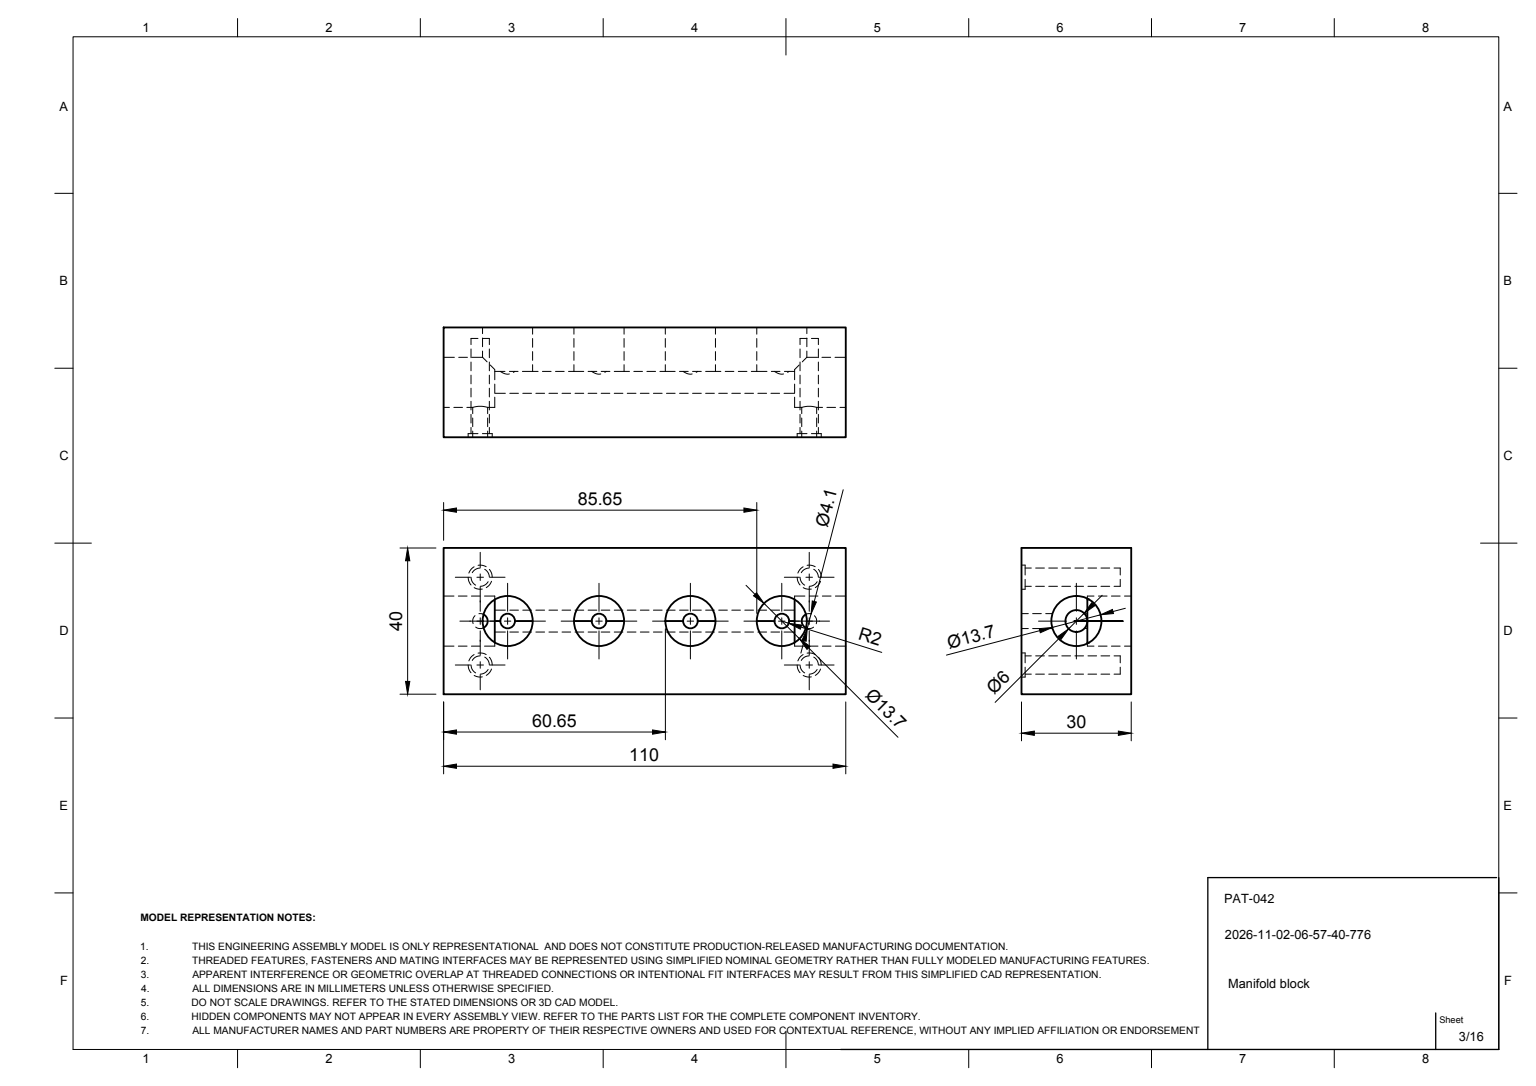
ISO-10303-21;
HEADER;
/* Generated by software containing ST-Developer
 * from STEP Tools, Inc. (www.steptools.com) 
 */

FILE_DESCRIPTION(
/* description */ ('Manifold and mounting hardware'),
/* implementation_level */ '2;1');

FILE_NAME(
/* name */ 'Manifold block.step',
/* time_stamp */ '2026-10-28T21:46:49-07:00',
/* author */ (''),
/* organization */ (''),
/* preprocessor_version */ 'ST-DEVELOPER v20.2',
/* originating_system */ 'Autodesk Translation Framework v15.17.0.0',
/* authorisation */ '');

FILE_SCHEMA (('AUTOMOTIVE_DESIGN { 1 0 10303 214 3 1 1 }'));
ENDSEC;

DATA;
#10=MECHANICAL_DESIGN_GEOMETRIC_PRESENTATION_REPRESENTATION('',(#150),#5638);
#122=SHAPE_REPRESENTATION_RELATIONSHIP('SRR','None',#5701,#136);
#136=ADVANCED_BREP_SHAPE_REPRESENTATION('',(#164),#5623);
#150=STYLED_ITEM('',(#5839),#164);
#164=MANIFOLD_SOLID_BREP('Body1',#3140);
#178=FACE_BOUND('',#528,.T.);
#179=FACE_BOUND('',#531,.T.);
#180=FACE_BOUND('',#539,.T.);
#181=FACE_BOUND('',#542,.T.);
#182=FACE_BOUND('',#545,.T.);
#183=FACE_BOUND('',#546,.T.);
#184=FACE_BOUND('',#555,.T.);
#185=FACE_BOUND('',#558,.T.);
#186=FACE_BOUND('',#560,.T.);
#187=FACE_BOUND('',#561,.T.);
#188=FACE_BOUND('',#562,.T.);
#189=FACE_BOUND('',#563,.T.);
#190=FACE_BOUND('',#565,.T.);
#191=FACE_BOUND('',#566,.T.);
#192=FACE_BOUND('',#567,.T.);
#193=FACE_BOUND('',#568,.T.);
#194=FACE_BOUND('',#569,.T.);
#195=FACE_BOUND('',#570,.T.);
#253=B_SPLINE_CURVE_WITH_KNOTS('',3,(#4697,#4698,#4699,#4700,#4701,#4702,
#4703,#4704,#4705,#4706),.UNSPECIFIED.,.F.,.F.,(4,2,2,2,4),(0.,0.0777490769060827,
0.155498153812165,0.233224303462309,0.310950453112452),.UNSPECIFIED.);
#254=B_SPLINE_CURVE_WITH_KNOTS('',3,(#4707,#4708,#4709,#4710,#4711,#4712,
#4713,#4714,#4715,#4716,#4717,#4718,#4719,#4720,#4721,#4722,#4723,#4724,
#4725,#4726,#4727,#4728,#4729,#4730,#4731,#4732),.UNSPECIFIED.,.F.,.F.,
(4,2,2,2,2,2,2,2,2,2,2,2,4),(0.310950453112452,0.388676602762596,0.466402752412739,
0.544151829318822,0.621900906224905,0.699649983130987,0.77739906003707,
0.855125209687213,0.932851359337357,1.0105775089875,1.08830365863764,1.16605273554373,
1.24380181244981),.UNSPECIFIED.);
#255=B_SPLINE_CURVE_WITH_KNOTS('',3,(#4767,#4768,#4769,#4770,#4771,#4772,
#4773,#4774,#4775,#4776),.UNSPECIFIED.,.F.,.F.,(4,2,2,2,4),(0.,0.0777490769060827,
0.155498153812165,0.233224303462309,0.310950453112452),.UNSPECIFIED.);
#256=B_SPLINE_CURVE_WITH_KNOTS('',3,(#4777,#4778,#4779,#4780,#4781,#4782,
#4783,#4784,#4785,#4786,#4787,#4788,#4789,#4790,#4791,#4792,#4793,#4794,
#4795,#4796,#4797,#4798,#4799,#4800,#4801,#4802),.UNSPECIFIED.,.F.,.F.,
(4,2,2,2,2,2,2,2,2,2,2,2,4),(0.310950453112452,0.388676602762596,0.466402752412739,
0.544151829318822,0.621900906224905,0.699649983130987,0.77739906003707,
0.855125209687213,0.932851359337357,1.0105775089875,1.08830365863764,1.16605273554373,
1.24380181244981),.UNSPECIFIED.);
#257=ELLIPSE('',#3314,0.96873629022557,0.685);
#258=ELLIPSE('',#3315,0.96873629022557,0.685);
#259=ELLIPSE('',#3316,0.96873629022557,0.685);
#260=ELLIPSE('',#3318,0.96873629022557,0.685);
#261=ELLIPSE('',#3325,0.96873629022557,0.685);
#262=ELLIPSE('',#3327,0.96873629022557,0.685);
#263=ELLIPSE('',#3329,0.96873629022557,0.685);
#264=ELLIPSE('',#3330,0.96873629022557,0.685);
#265=ELLIPSE('',#3371,0.96873629022557,0.685);
#266=ELLIPSE('',#3372,0.96873629022557,0.685);
#267=ELLIPSE('',#3373,0.96873629022557,0.685);
#268=ELLIPSE('',#3374,0.96873629022557,0.685);
#269=ELLIPSE('',#3376,0.96873629022557,0.685);
#270=ELLIPSE('',#3377,0.96873629022557,0.685);
#271=ELLIPSE('',#3378,0.96873629022557,0.685);
#272=ELLIPSE('',#3379,0.96873629022557,0.685);
#273=CYLINDRICAL_SURFACE('',#3313,0.685);
#274=CYLINDRICAL_SURFACE('',#3324,0.685);
#275=CYLINDRICAL_SURFACE('',#3332,0.205);
#276=CYLINDRICAL_SURFACE('',#3334,0.25);
#277=CYLINDRICAL_SURFACE('',#3338,0.25);
#278=CYLINDRICAL_SURFACE('',#3342,0.33);
#279=CYLINDRICAL_SURFACE('',#3346,0.33);
#280=CYLINDRICAL_SURFACE('',#3350,0.205);
#281=CYLINDRICAL_SURFACE('',#3352,0.25);
#282=CYLINDRICAL_SURFACE('',#3356,0.25);
#283=CYLINDRICAL_SURFACE('',#3360,0.33);
#284=CYLINDRICAL_SURFACE('',#3364,0.33);
#285=CYLINDRICAL_SURFACE('',#3369,0.685);
#286=CYLINDRICAL_SURFACE('',#3382,0.685);
#287=CYLINDRICAL_SURFACE('',#3386,0.685);
#330=FACE_OUTER_BOUND('',#516,.T.);
#331=FACE_OUTER_BOUND('',#517,.T.);
#332=FACE_OUTER_BOUND('',#518,.T.);
#333=FACE_OUTER_BOUND('',#519,.T.);
#334=FACE_OUTER_BOUND('',#520,.T.);
#335=FACE_OUTER_BOUND('',#521,.T.);
#336=FACE_OUTER_BOUND('',#522,.T.);
#337=FACE_OUTER_BOUND('',#523,.T.);
#338=FACE_OUTER_BOUND('',#524,.T.);
#339=FACE_OUTER_BOUND('',#525,.T.);
#340=FACE_OUTER_BOUND('',#526,.T.);
#341=FACE_OUTER_BOUND('',#527,.T.);
#342=FACE_OUTER_BOUND('',#529,.T.);
#343=FACE_OUTER_BOUND('',#530,.T.);
#344=FACE_OUTER_BOUND('',#532,.T.);
#345=FACE_OUTER_BOUND('',#533,.T.);
#346=FACE_OUTER_BOUND('',#534,.T.);
#347=FACE_OUTER_BOUND('',#535,.T.);
#348=FACE_OUTER_BOUND('',#536,.T.);
#349=FACE_OUTER_BOUND('',#537,.T.);
#350=FACE_OUTER_BOUND('',#538,.T.);
#351=FACE_OUTER_BOUND('',#540,.T.);
#352=FACE_OUTER_BOUND('',#541,.T.);
#353=FACE_OUTER_BOUND('',#543,.T.);
#354=FACE_OUTER_BOUND('',#544,.T.);
#355=FACE_OUTER_BOUND('',#547,.T.);
#356=FACE_OUTER_BOUND('',#548,.T.);
#357=FACE_OUTER_BOUND('',#549,.T.);
#358=FACE_OUTER_BOUND('',#550,.T.);
#359=FACE_OUTER_BOUND('',#551,.T.);
#360=FACE_OUTER_BOUND('',#552,.T.);
#361=FACE_OUTER_BOUND('',#553,.T.);
#362=FACE_OUTER_BOUND('',#554,.T.);
#363=FACE_OUTER_BOUND('',#556,.T.);
#364=FACE_OUTER_BOUND('',#557,.T.);
#365=FACE_OUTER_BOUND('',#559,.T.);
#366=FACE_OUTER_BOUND('',#564,.T.);
#516=EDGE_LOOP('',(#2044,#2045));
#517=EDGE_LOOP('',(#2046,#2047,#2048,#2049,#2050,#2051,#2052,#2053,#2054));
#518=EDGE_LOOP('',(#2055,#2056));
#519=EDGE_LOOP('',(#2057,#2058));
#520=EDGE_LOOP('',(#2059,#2060,#2061,#2062,#2063,#2064,#2065,#2066,#2067));
#521=EDGE_LOOP('',(#2068,#2069,#2070,#2071,#2072));
#522=EDGE_LOOP('',(#2073,#2074,#2075,#2076));
#523=EDGE_LOOP('',(#2077));
#524=EDGE_LOOP('',(#2078,#2079,#2080,#2081));
#525=EDGE_LOOP('',(#2082));
#526=EDGE_LOOP('',(#2083,#2084,#2085,#2086));
#527=EDGE_LOOP('',(#2087));
#528=EDGE_LOOP('',(#2088));
#529=EDGE_LOOP('',(#2089,#2090,#2091,#2092));
#530=EDGE_LOOP('',(#2093));
#531=EDGE_LOOP('',(#2094));
#532=EDGE_LOOP('',(#2095,#2096,#2097,#2098,#2099));
#533=EDGE_LOOP('',(#2100,#2101,#2102,#2103));
#534=EDGE_LOOP('',(#2104));
#535=EDGE_LOOP('',(#2105,#2106,#2107,#2108));
#536=EDGE_LOOP('',(#2109));
#537=EDGE_LOOP('',(#2110,#2111,#2112,#2113));
#538=EDGE_LOOP('',(#2114));
#539=EDGE_LOOP('',(#2115));
#540=EDGE_LOOP('',(#2116,#2117,#2118,#2119));
#541=EDGE_LOOP('',(#2120));
#542=EDGE_LOOP('',(#2121));
#543=EDGE_LOOP('',(#2122,#2123));
#544=EDGE_LOOP('',(#2124,#2125,#2126,#2127,#2128,#2129,#2130,#2131,#2132,
#2133,#2134,#2135,#2136,#2137,#2138,#2139,#2140,#2141,#2142,#2143,#2144,
#2145,#2146,#2147,#2148,#2149,#2150,#2151,#2152,#2153,#2154,#2155,#2156,
#2157,#2158,#2159));
#545=EDGE_LOOP('',(#2160,#2161));
#546=EDGE_LOOP('',(#2162,#2163));
#547=EDGE_LOOP('',(#2164,#2165));
#548=EDGE_LOOP('',(#2166,#2167,#2168,#2169,#2170,#2171,#2172,#2173,#2174));
#549=EDGE_LOOP('',(#2175,#2176));
#550=EDGE_LOOP('',(#2177,#2178,#2179,#2180,#2181,#2182,#2183,#2184,#2185));
#551=EDGE_LOOP('',(#2186,#2187));
#552=EDGE_LOOP('',(#2188,#2189));
#553=EDGE_LOOP('',(#2190,#2191,#2192,#2193));
#554=EDGE_LOOP('',(#2194,#2195,#2196,#2197));
#555=EDGE_LOOP('',(#2198));
#556=EDGE_LOOP('',(#2199,#2200,#2201,#2202));
#557=EDGE_LOOP('',(#2203,#2204,#2205,#2206));
#558=EDGE_LOOP('',(#2207));
#559=EDGE_LOOP('',(#2208,#2209,#2210,#2211));
#560=EDGE_LOOP('',(#2212));
#561=EDGE_LOOP('',(#2213));
#562=EDGE_LOOP('',(#2214));
#563=EDGE_LOOP('',(#2215));
#564=EDGE_LOOP('',(#2216,#2217,#2218,#2219));
#565=EDGE_LOOP('',(#2220));
#566=EDGE_LOOP('',(#2221));
#567=EDGE_LOOP('',(#2222));
#568=EDGE_LOOP('',(#2223));
#569=EDGE_LOOP('',(#2224));
#570=EDGE_LOOP('',(#2225));
#777=CIRCLE('',#3312,0.685);
#778=CIRCLE('',#3317,0.685);
#779=CIRCLE('',#3319,0.685);
#780=CIRCLE('',#3321,0.685);
#781=CIRCLE('',#3323,0.685);
#782=CIRCLE('',#3326,0.685);
#783=CIRCLE('',#3328,0.685);
#784=CIRCLE('',#3331,0.685);
#785=CIRCLE('',#3333,0.205);
#786=CIRCLE('',#3335,0.25);
#787=CIRCLE('',#3336,0.25);
#788=CIRCLE('',#3339,0.25);
#789=CIRCLE('',#3340,0.25);
#790=CIRCLE('',#3343,0.33);
#791=CIRCLE('',#3344,0.33);
#792=CIRCLE('',#3347,0.33);
#793=CIRCLE('',#3348,0.33);
#794=CIRCLE('',#3351,0.205);
#795=CIRCLE('',#3353,0.25);
#796=CIRCLE('',#3354,0.25);
#797=CIRCLE('',#3357,0.25);
#798=CIRCLE('',#3358,0.25);
#799=CIRCLE('',#3361,0.33);
#800=CIRCLE('',#3362,0.33);
#801=CIRCLE('',#3365,0.33);
#802=CIRCLE('',#3366,0.33);
#803=CIRCLE('',#3370,0.685);
#804=CIRCLE('',#3375,0.685);
#805=CIRCLE('',#3381,0.685);
#806=CIRCLE('',#3383,0.685);
#807=CIRCLE('',#3385,0.685);
#808=CIRCLE('',#3387,0.685);
#897=LINE('',#4650,#1144);
#898=LINE('',#4660,#1145);
#899=LINE('',#4668,#1146);
#900=LINE('',#4673,#1147);
#901=LINE('',#4680,#1148);
#902=LINE('',#4695,#1149);
#903=LINE('',#4737,#1150);
#904=LINE('',#4744,#1151);
#905=LINE('',#4751,#1152);
#906=LINE('',#4758,#1153);
#907=LINE('',#4765,#1154);
#908=LINE('',#4807,#1155);
#909=LINE('',#4814,#1156);
#910=LINE('',#4821,#1157);
#911=LINE('',#4828,#1158);
#912=LINE('',#4832,#1159);
#913=LINE('',#4836,#1160);
#914=LINE('',#4837,#1161);
#915=LINE('',#4839,#1162);
#916=LINE('',#4843,#1163);
#917=LINE('',#4847,#1164);
#918=LINE('',#4851,#1165);
#919=LINE('',#4854,#1166);
#920=LINE('',#4856,#1167);
#921=LINE('',#4862,#1168);
#922=LINE('',#4867,#1169);
#923=LINE('',#4873,#1170);
#924=LINE('',#4880,#1171);
#925=LINE('',#4882,#1172);
#926=LINE('',#4884,#1173);
#927=LINE('',#4885,#1174);
#928=LINE('',#4888,#1175);
#929=LINE('',#4890,#1176);
#930=LINE('',#4891,#1177);
#931=LINE('',#4894,#1178);
#932=LINE('',#4896,#1179);
#933=LINE('',#4897,#1180);
#934=LINE('',#4899,#1181);
#935=LINE('',#4900,#1182);
#1144=VECTOR('',#3678,1.);
#1145=VECTOR('',#3689,0.685);
#1146=VECTOR('',#3698,1.);
#1147=VECTOR('',#3703,1.);
#1148=VECTOR('',#3710,0.685);
#1149=VECTOR('',#3727,0.205);
#1150=VECTOR('',#3732,0.25);
#1151=VECTOR('',#3741,0.25);
#1152=VECTOR('',#3750,0.33);
#1153=VECTOR('',#3759,0.33);
#1154=VECTOR('',#3768,0.205);
#1155=VECTOR('',#3773,0.25);
#1156=VECTOR('',#3782,0.25);
#1157=VECTOR('',#3791,0.33);
#1158=VECTOR('',#3800,0.33);
#1159=VECTOR('',#3807,1.);
#1160=VECTOR('',#3812,0.685);
#1161=VECTOR('',#3813,1.);
#1162=VECTOR('',#3814,0.685);
#1163=VECTOR('',#3817,1.);
#1164=VECTOR('',#3820,0.685);
#1165=VECTOR('',#3823,1.);
#1166=VECTOR('',#3826,0.685);
#1167=VECTOR('',#3827,0.685);
#1168=VECTOR('',#3838,1.);
#1169=VECTOR('',#3845,0.685);
#1170=VECTOR('',#3854,0.685);
#1171=VECTOR('',#3863,1.);
#1172=VECTOR('',#3864,1.);
#1173=VECTOR('',#3865,1.);
#1174=VECTOR('',#3866,1.);
#1175=VECTOR('',#3869,1.);
#1176=VECTOR('',#3870,1.);
#1177=VECTOR('',#3871,1.);
#1178=VECTOR('',#3874,1.);
#1179=VECTOR('',#3875,1.);
#1180=VECTOR('',#3876,1.);
#1181=VECTOR('',#3879,1.);
#1182=VECTOR('',#3880,1.);
#1391=VERTEX_POINT('',#4648);
#1392=VERTEX_POINT('',#4649);
#1393=VERTEX_POINT('',#4653);
#1394=VERTEX_POINT('',#4654);
#1395=VERTEX_POINT('',#4657);
#1396=VERTEX_POINT('',#4659);
#1397=VERTEX_POINT('',#4662);
#1398=VERTEX_POINT('',#4666);
#1399=VERTEX_POINT('',#4667);
#1400=VERTEX_POINT('',#4671);
#1401=VERTEX_POINT('',#4672);
#1402=VERTEX_POINT('',#4676);
#1403=VERTEX_POINT('',#4677);
#1404=VERTEX_POINT('',#4679);
#1405=VERTEX_POINT('',#4682);
#1406=VERTEX_POINT('',#4684);
#1407=VERTEX_POINT('',#4686);
#1408=VERTEX_POINT('',#4688);
#1409=VERTEX_POINT('',#4692);
#1410=VERTEX_POINT('',#4694);
#1411=VERTEX_POINT('',#4696);
#1412=VERTEX_POINT('',#4734);
#1413=VERTEX_POINT('',#4736);
#1414=VERTEX_POINT('',#4741);
#1415=VERTEX_POINT('',#4743);
#1416=VERTEX_POINT('',#4748);
#1417=VERTEX_POINT('',#4750);
#1418=VERTEX_POINT('',#4755);
#1419=VERTEX_POINT('',#4757);
#1420=VERTEX_POINT('',#4762);
#1421=VERTEX_POINT('',#4764);
#1422=VERTEX_POINT('',#4766);
#1423=VERTEX_POINT('',#4804);
#1424=VERTEX_POINT('',#4806);
#1425=VERTEX_POINT('',#4811);
#1426=VERTEX_POINT('',#4813);
#1427=VERTEX_POINT('',#4818);
#1428=VERTEX_POINT('',#4820);
#1429=VERTEX_POINT('',#4825);
#1430=VERTEX_POINT('',#4827);
#1431=VERTEX_POINT('',#4834);
#1432=VERTEX_POINT('',#4838);
#1433=VERTEX_POINT('',#4840);
#1434=VERTEX_POINT('',#4842);
#1435=VERTEX_POINT('',#4844);
#1436=VERTEX_POINT('',#4846);
#1437=VERTEX_POINT('',#4848);
#1438=VERTEX_POINT('',#4850);
#1439=VERTEX_POINT('',#4852);
#1440=VERTEX_POINT('',#4855);
#1441=VERTEX_POINT('',#4866);
#1442=VERTEX_POINT('',#4872);
#1443=VERTEX_POINT('',#4878);
#1444=VERTEX_POINT('',#4879);
#1445=VERTEX_POINT('',#4881);
#1446=VERTEX_POINT('',#4883);
#1447=VERTEX_POINT('',#4887);
#1448=VERTEX_POINT('',#4889);
#1449=VERTEX_POINT('',#4893);
#1450=VERTEX_POINT('',#4895);
#1651=EDGE_CURVE('',#1391,#1392,#897,.T.);
#1652=EDGE_CURVE('',#1392,#1391,#777,.T.);
#1653=EDGE_CURVE('',#1393,#1394,#257,.T.);
#1654=EDGE_CURVE('',#1394,#1391,#258,.T.);
#1655=EDGE_CURVE('',#1392,#1395,#259,.T.);
#1656=EDGE_CURVE('',#1395,#1396,#898,.T.);
#1657=EDGE_CURVE('',#1396,#1396,#778,.T.);
#1658=EDGE_CURVE('',#1395,#1397,#260,.T.);
#1659=EDGE_CURVE('',#1393,#1397,#779,.T.);
#1660=EDGE_CURVE('',#1398,#1399,#899,.T.);
#1661=EDGE_CURVE('',#1399,#1398,#780,.T.);
#1662=EDGE_CURVE('',#1400,#1401,#900,.T.);
#1663=EDGE_CURVE('',#1401,#1400,#781,.T.);
#1664=EDGE_CURVE('',#1402,#1403,#261,.T.);
#1665=EDGE_CURVE('',#1403,#1404,#901,.T.);
#1666=EDGE_CURVE('',#1404,#1404,#782,.T.);
#1667=EDGE_CURVE('',#1403,#1405,#262,.T.);
#1668=EDGE_CURVE('',#1406,#1405,#783,.T.);
#1669=EDGE_CURVE('',#1406,#1407,#263,.T.);
#1670=EDGE_CURVE('',#1407,#1408,#264,.T.);
#1671=EDGE_CURVE('',#1402,#1408,#784,.T.);
#1672=EDGE_CURVE('',#1409,#1409,#785,.T.);
#1673=EDGE_CURVE('',#1409,#1410,#902,.T.);
#1674=EDGE_CURVE('',#1411,#1410,#253,.T.);
#1675=EDGE_CURVE('',#1410,#1411,#254,.T.);
#1676=EDGE_CURVE('',#1412,#1412,#786,.T.);
#1677=EDGE_CURVE('',#1412,#1413,#903,.T.);
#1678=EDGE_CURVE('',#1413,#1413,#787,.T.);
#1679=EDGE_CURVE('',#1414,#1414,#788,.T.);
#1680=EDGE_CURVE('',#1414,#1415,#904,.T.);
#1681=EDGE_CURVE('',#1415,#1415,#789,.T.);
#1682=EDGE_CURVE('',#1416,#1416,#790,.T.);
#1683=EDGE_CURVE('',#1416,#1417,#905,.T.);
#1684=EDGE_CURVE('',#1417,#1417,#791,.T.);
#1685=EDGE_CURVE('',#1418,#1418,#792,.T.);
#1686=EDGE_CURVE('',#1418,#1419,#906,.T.);
#1687=EDGE_CURVE('',#1419,#1419,#793,.T.);
#1688=EDGE_CURVE('',#1420,#1420,#794,.T.);
#1689=EDGE_CURVE('',#1420,#1421,#907,.T.);
#1690=EDGE_CURVE('',#1422,#1421,#255,.T.);
#1691=EDGE_CURVE('',#1421,#1422,#256,.T.);
#1692=EDGE_CURVE('',#1423,#1423,#795,.T.);
#1693=EDGE_CURVE('',#1423,#1424,#908,.T.);
#1694=EDGE_CURVE('',#1424,#1424,#796,.T.);
#1695=EDGE_CURVE('',#1425,#1425,#797,.T.);
#1696=EDGE_CURVE('',#1425,#1426,#909,.T.);
#1697=EDGE_CURVE('',#1426,#1426,#798,.T.);
#1698=EDGE_CURVE('',#1427,#1427,#799,.T.);
#1699=EDGE_CURVE('',#1427,#1428,#910,.T.);
#1700=EDGE_CURVE('',#1428,#1428,#800,.T.);
#1701=EDGE_CURVE('',#1429,#1429,#801,.T.);
#1702=EDGE_CURVE('',#1429,#1430,#911,.T.);
#1703=EDGE_CURVE('',#1430,#1430,#802,.T.);
#1704=EDGE_CURVE('',#1397,#1393,#912,.T.);
#1705=EDGE_CURVE('',#1431,#1431,#803,.T.);
#1706=EDGE_CURVE('',#1431,#1403,#913,.T.);
#1707=EDGE_CURVE('',#1408,#1402,#914,.T.);
#1708=EDGE_CURVE('',#1407,#1432,#915,.T.);
#1709=EDGE_CURVE('',#1433,#1432,#265,.T.);
#1710=EDGE_CURVE('',#1434,#1433,#916,.T.);
#1711=EDGE_CURVE('',#1435,#1434,#266,.T.);
#1712=EDGE_CURVE('',#1435,#1436,#917,.T.);
#1713=EDGE_CURVE('',#1437,#1436,#267,.T.);
#1714=EDGE_CURVE('',#1438,#1437,#918,.T.);
#1715=EDGE_CURVE('',#1439,#1438,#268,.T.);
#1716=EDGE_CURVE('',#1439,#1395,#919,.T.);
#1717=EDGE_CURVE('',#1394,#1440,#920,.T.);
#1718=EDGE_CURVE('',#1440,#1440,#804,.T.);
#1719=EDGE_CURVE('',#1399,#1439,#269,.T.);
#1720=EDGE_CURVE('',#1436,#1398,#270,.T.);
#1721=EDGE_CURVE('',#1401,#1435,#271,.T.);
#1722=EDGE_CURVE('',#1432,#1400,#272,.T.);
#1723=EDGE_CURVE('',#1405,#1406,#921,.T.);
#1724=EDGE_CURVE('',#1437,#1438,#805,.T.);
#1725=EDGE_CURVE('',#1436,#1441,#922,.T.);
#1726=EDGE_CURVE('',#1441,#1441,#806,.T.);
#1727=EDGE_CURVE('',#1433,#1434,#807,.T.);
#1728=EDGE_CURVE('',#1432,#1442,#923,.T.);
#1729=EDGE_CURVE('',#1442,#1442,#808,.T.);
#1730=EDGE_CURVE('',#1443,#1444,#924,.T.);
#1731=EDGE_CURVE('',#1444,#1445,#925,.T.);
#1732=EDGE_CURVE('',#1446,#1445,#926,.T.);
#1733=EDGE_CURVE('',#1443,#1446,#927,.T.);
#1734=EDGE_CURVE('',#1447,#1443,#928,.T.);
#1735=EDGE_CURVE('',#1448,#1446,#929,.T.);
#1736=EDGE_CURVE('',#1447,#1448,#930,.T.);
#1737=EDGE_CURVE('',#1449,#1447,#931,.T.);
#1738=EDGE_CURVE('',#1450,#1448,#932,.T.);
#1739=EDGE_CURVE('',#1449,#1450,#933,.T.);
#1740=EDGE_CURVE('',#1444,#1449,#934,.T.);
#1741=EDGE_CURVE('',#1445,#1450,#935,.T.);
#2044=ORIENTED_EDGE('',*,*,#1651,.T.);
#2045=ORIENTED_EDGE('',*,*,#1652,.T.);
#2046=ORIENTED_EDGE('',*,*,#1653,.T.);
#2047=ORIENTED_EDGE('',*,*,#1654,.T.);
#2048=ORIENTED_EDGE('',*,*,#1652,.F.);
#2049=ORIENTED_EDGE('',*,*,#1655,.T.);
#2050=ORIENTED_EDGE('',*,*,#1656,.T.);
#2051=ORIENTED_EDGE('',*,*,#1657,.F.);
#2052=ORIENTED_EDGE('',*,*,#1656,.F.);
#2053=ORIENTED_EDGE('',*,*,#1658,.T.);
#2054=ORIENTED_EDGE('',*,*,#1659,.F.);
#2055=ORIENTED_EDGE('',*,*,#1660,.T.);
#2056=ORIENTED_EDGE('',*,*,#1661,.T.);
#2057=ORIENTED_EDGE('',*,*,#1662,.T.);
#2058=ORIENTED_EDGE('',*,*,#1663,.T.);
#2059=ORIENTED_EDGE('',*,*,#1664,.T.);
#2060=ORIENTED_EDGE('',*,*,#1665,.T.);
#2061=ORIENTED_EDGE('',*,*,#1666,.F.);
#2062=ORIENTED_EDGE('',*,*,#1665,.F.);
#2063=ORIENTED_EDGE('',*,*,#1667,.T.);
#2064=ORIENTED_EDGE('',*,*,#1668,.F.);
#2065=ORIENTED_EDGE('',*,*,#1669,.T.);
#2066=ORIENTED_EDGE('',*,*,#1670,.T.);
#2067=ORIENTED_EDGE('',*,*,#1671,.F.);
#2068=ORIENTED_EDGE('',*,*,#1672,.F.);
#2069=ORIENTED_EDGE('',*,*,#1673,.T.);
#2070=ORIENTED_EDGE('',*,*,#1674,.F.);
#2071=ORIENTED_EDGE('',*,*,#1675,.F.);
#2072=ORIENTED_EDGE('',*,*,#1673,.F.);
#2073=ORIENTED_EDGE('',*,*,#1676,.F.);
#2074=ORIENTED_EDGE('',*,*,#1677,.T.);
#2075=ORIENTED_EDGE('',*,*,#1678,.T.);
#2076=ORIENTED_EDGE('',*,*,#1677,.F.);
#2077=ORIENTED_EDGE('',*,*,#1678,.F.);
#2078=ORIENTED_EDGE('',*,*,#1679,.F.);
#2079=ORIENTED_EDGE('',*,*,#1680,.T.);
#2080=ORIENTED_EDGE('',*,*,#1681,.T.);
#2081=ORIENTED_EDGE('',*,*,#1680,.F.);
#2082=ORIENTED_EDGE('',*,*,#1681,.F.);
#2083=ORIENTED_EDGE('',*,*,#1682,.F.);
#2084=ORIENTED_EDGE('',*,*,#1683,.T.);
#2085=ORIENTED_EDGE('',*,*,#1684,.T.);
#2086=ORIENTED_EDGE('',*,*,#1683,.F.);
#2087=ORIENTED_EDGE('',*,*,#1684,.F.);
#2088=ORIENTED_EDGE('',*,*,#1676,.T.);
#2089=ORIENTED_EDGE('',*,*,#1685,.F.);
#2090=ORIENTED_EDGE('',*,*,#1686,.T.);
#2091=ORIENTED_EDGE('',*,*,#1687,.T.);
#2092=ORIENTED_EDGE('',*,*,#1686,.F.);
#2093=ORIENTED_EDGE('',*,*,#1687,.F.);
#2094=ORIENTED_EDGE('',*,*,#1679,.T.);
#2095=ORIENTED_EDGE('',*,*,#1688,.F.);
#2096=ORIENTED_EDGE('',*,*,#1689,.T.);
#2097=ORIENTED_EDGE('',*,*,#1690,.F.);
#2098=ORIENTED_EDGE('',*,*,#1691,.F.);
#2099=ORIENTED_EDGE('',*,*,#1689,.F.);
#2100=ORIENTED_EDGE('',*,*,#1692,.F.);
#2101=ORIENTED_EDGE('',*,*,#1693,.T.);
#2102=ORIENTED_EDGE('',*,*,#1694,.T.);
#2103=ORIENTED_EDGE('',*,*,#1693,.F.);
#2104=ORIENTED_EDGE('',*,*,#1694,.F.);
#2105=ORIENTED_EDGE('',*,*,#1695,.F.);
#2106=ORIENTED_EDGE('',*,*,#1696,.T.);
#2107=ORIENTED_EDGE('',*,*,#1697,.T.);
#2108=ORIENTED_EDGE('',*,*,#1696,.F.);
#2109=ORIENTED_EDGE('',*,*,#1697,.F.);
#2110=ORIENTED_EDGE('',*,*,#1698,.F.);
#2111=ORIENTED_EDGE('',*,*,#1699,.T.);
#2112=ORIENTED_EDGE('',*,*,#1700,.T.);
#2113=ORIENTED_EDGE('',*,*,#1699,.F.);
#2114=ORIENTED_EDGE('',*,*,#1700,.F.);
#2115=ORIENTED_EDGE('',*,*,#1692,.T.);
#2116=ORIENTED_EDGE('',*,*,#1701,.F.);
#2117=ORIENTED_EDGE('',*,*,#1702,.T.);
#2118=ORIENTED_EDGE('',*,*,#1703,.T.);
#2119=ORIENTED_EDGE('',*,*,#1702,.F.);
#2120=ORIENTED_EDGE('',*,*,#1703,.F.);
#2121=ORIENTED_EDGE('',*,*,#1695,.T.);
#2122=ORIENTED_EDGE('',*,*,#1704,.T.);
#2123=ORIENTED_EDGE('',*,*,#1659,.T.);
#2124=ORIENTED_EDGE('',*,*,#1705,.F.);
#2125=ORIENTED_EDGE('',*,*,#1706,.T.);
#2126=ORIENTED_EDGE('',*,*,#1664,.F.);
#2127=ORIENTED_EDGE('',*,*,#1707,.F.);
#2128=ORIENTED_EDGE('',*,*,#1670,.F.);
#2129=ORIENTED_EDGE('',*,*,#1708,.T.);
#2130=ORIENTED_EDGE('',*,*,#1709,.F.);
#2131=ORIENTED_EDGE('',*,*,#1710,.F.);
#2132=ORIENTED_EDGE('',*,*,#1711,.F.);
#2133=ORIENTED_EDGE('',*,*,#1712,.T.);
#2134=ORIENTED_EDGE('',*,*,#1713,.F.);
#2135=ORIENTED_EDGE('',*,*,#1714,.F.);
#2136=ORIENTED_EDGE('',*,*,#1715,.F.);
#2137=ORIENTED_EDGE('',*,*,#1716,.T.);
#2138=ORIENTED_EDGE('',*,*,#1655,.F.);
#2139=ORIENTED_EDGE('',*,*,#1651,.F.);
#2140=ORIENTED_EDGE('',*,*,#1654,.F.);
#2141=ORIENTED_EDGE('',*,*,#1717,.T.);
#2142=ORIENTED_EDGE('',*,*,#1718,.F.);
#2143=ORIENTED_EDGE('',*,*,#1717,.F.);
#2144=ORIENTED_EDGE('',*,*,#1653,.F.);
#2145=ORIENTED_EDGE('',*,*,#1704,.F.);
#2146=ORIENTED_EDGE('',*,*,#1658,.F.);
#2147=ORIENTED_EDGE('',*,*,#1716,.F.);
#2148=ORIENTED_EDGE('',*,*,#1719,.F.);
#2149=ORIENTED_EDGE('',*,*,#1660,.F.);
#2150=ORIENTED_EDGE('',*,*,#1720,.F.);
#2151=ORIENTED_EDGE('',*,*,#1712,.F.);
#2152=ORIENTED_EDGE('',*,*,#1721,.F.);
#2153=ORIENTED_EDGE('',*,*,#1662,.F.);
#2154=ORIENTED_EDGE('',*,*,#1722,.F.);
#2155=ORIENTED_EDGE('',*,*,#1708,.F.);
#2156=ORIENTED_EDGE('',*,*,#1669,.F.);
#2157=ORIENTED_EDGE('',*,*,#1723,.F.);
#2158=ORIENTED_EDGE('',*,*,#1667,.F.);
#2159=ORIENTED_EDGE('',*,*,#1706,.F.);
#2160=ORIENTED_EDGE('',*,*,#1690,.T.);
#2161=ORIENTED_EDGE('',*,*,#1691,.T.);
#2162=ORIENTED_EDGE('',*,*,#1674,.T.);
#2163=ORIENTED_EDGE('',*,*,#1675,.T.);
#2164=ORIENTED_EDGE('',*,*,#1714,.T.);
#2165=ORIENTED_EDGE('',*,*,#1724,.T.);
#2166=ORIENTED_EDGE('',*,*,#1713,.T.);
#2167=ORIENTED_EDGE('',*,*,#1725,.T.);
#2168=ORIENTED_EDGE('',*,*,#1726,.F.);
#2169=ORIENTED_EDGE('',*,*,#1725,.F.);
#2170=ORIENTED_EDGE('',*,*,#1720,.T.);
#2171=ORIENTED_EDGE('',*,*,#1661,.F.);
#2172=ORIENTED_EDGE('',*,*,#1719,.T.);
#2173=ORIENTED_EDGE('',*,*,#1715,.T.);
#2174=ORIENTED_EDGE('',*,*,#1724,.F.);
#2175=ORIENTED_EDGE('',*,*,#1710,.T.);
#2176=ORIENTED_EDGE('',*,*,#1727,.T.);
#2177=ORIENTED_EDGE('',*,*,#1709,.T.);
#2178=ORIENTED_EDGE('',*,*,#1728,.T.);
#2179=ORIENTED_EDGE('',*,*,#1729,.F.);
#2180=ORIENTED_EDGE('',*,*,#1728,.F.);
#2181=ORIENTED_EDGE('',*,*,#1722,.T.);
#2182=ORIENTED_EDGE('',*,*,#1663,.F.);
#2183=ORIENTED_EDGE('',*,*,#1721,.T.);
#2184=ORIENTED_EDGE('',*,*,#1711,.T.);
#2185=ORIENTED_EDGE('',*,*,#1727,.F.);
#2186=ORIENTED_EDGE('',*,*,#1707,.T.);
#2187=ORIENTED_EDGE('',*,*,#1671,.T.);
#2188=ORIENTED_EDGE('',*,*,#1723,.T.);
#2189=ORIENTED_EDGE('',*,*,#1668,.T.);
#2190=ORIENTED_EDGE('',*,*,#1730,.T.);
#2191=ORIENTED_EDGE('',*,*,#1731,.T.);
#2192=ORIENTED_EDGE('',*,*,#1732,.F.);
#2193=ORIENTED_EDGE('',*,*,#1733,.F.);
#2194=ORIENTED_EDGE('',*,*,#1734,.T.);
#2195=ORIENTED_EDGE('',*,*,#1733,.T.);
#2196=ORIENTED_EDGE('',*,*,#1735,.F.);
#2197=ORIENTED_EDGE('',*,*,#1736,.F.);
#2198=ORIENTED_EDGE('',*,*,#1718,.T.);
#2199=ORIENTED_EDGE('',*,*,#1737,.T.);
#2200=ORIENTED_EDGE('',*,*,#1736,.T.);
#2201=ORIENTED_EDGE('',*,*,#1738,.F.);
#2202=ORIENTED_EDGE('',*,*,#1739,.F.);
#2203=ORIENTED_EDGE('',*,*,#1740,.T.);
#2204=ORIENTED_EDGE('',*,*,#1739,.T.);
#2205=ORIENTED_EDGE('',*,*,#1741,.F.);
#2206=ORIENTED_EDGE('',*,*,#1731,.F.);
#2207=ORIENTED_EDGE('',*,*,#1705,.T.);
#2208=ORIENTED_EDGE('',*,*,#1741,.T.);
#2209=ORIENTED_EDGE('',*,*,#1738,.T.);
#2210=ORIENTED_EDGE('',*,*,#1735,.T.);
#2211=ORIENTED_EDGE('',*,*,#1732,.T.);
#2212=ORIENTED_EDGE('',*,*,#1657,.T.);
#2213=ORIENTED_EDGE('',*,*,#1726,.T.);
#2214=ORIENTED_EDGE('',*,*,#1729,.T.);
#2215=ORIENTED_EDGE('',*,*,#1666,.T.);
#2216=ORIENTED_EDGE('',*,*,#1740,.F.);
#2217=ORIENTED_EDGE('',*,*,#1730,.F.);
#2218=ORIENTED_EDGE('',*,*,#1734,.F.);
#2219=ORIENTED_EDGE('',*,*,#1737,.F.);
#2220=ORIENTED_EDGE('',*,*,#1672,.T.);
#2221=ORIENTED_EDGE('',*,*,#1682,.T.);
#2222=ORIENTED_EDGE('',*,*,#1685,.T.);
#2223=ORIENTED_EDGE('',*,*,#1688,.T.);
#2224=ORIENTED_EDGE('',*,*,#1698,.T.);
#2225=ORIENTED_EDGE('',*,*,#1701,.T.);
#2830=PLANE('',#3311);
#2831=PLANE('',#3320);
#2832=PLANE('',#3322);
#2833=PLANE('',#3337);
#2834=PLANE('',#3341);
#2835=PLANE('',#3345);
#2836=PLANE('',#3349);
#2837=PLANE('',#3355);
#2838=PLANE('',#3359);
#2839=PLANE('',#3363);
#2840=PLANE('',#3367);
#2841=PLANE('',#3368);
#2842=PLANE('',#3380);
#2843=PLANE('',#3384);
#2844=PLANE('',#3388);
#2845=PLANE('',#3389);
#2846=PLANE('',#3390);
#2847=PLANE('',#3391);
#2848=PLANE('',#3392);
#2849=PLANE('',#3393);
#2850=PLANE('',#3394);
#2851=PLANE('',#3395);
#2954=ADVANCED_FACE('',(#330),#2830,.T.);
#2955=ADVANCED_FACE('',(#331),#273,.F.);
#2956=ADVANCED_FACE('',(#332),#2831,.T.);
#2957=ADVANCED_FACE('',(#333),#2832,.T.);
#2958=ADVANCED_FACE('',(#334),#274,.F.);
#2959=ADVANCED_FACE('',(#335),#275,.F.);
#2960=ADVANCED_FACE('',(#336),#276,.F.);
#2961=ADVANCED_FACE('',(#337),#2833,.F.);
#2962=ADVANCED_FACE('',(#338),#277,.F.);
#2963=ADVANCED_FACE('',(#339),#2834,.F.);
#2964=ADVANCED_FACE('',(#340),#278,.F.);
#2965=ADVANCED_FACE('',(#341,#178),#2835,.F.);
#2966=ADVANCED_FACE('',(#342),#279,.F.);
#2967=ADVANCED_FACE('',(#343,#179),#2836,.F.);
#2968=ADVANCED_FACE('',(#344),#280,.F.);
#2969=ADVANCED_FACE('',(#345),#281,.F.);
#2970=ADVANCED_FACE('',(#346),#2837,.F.);
#2971=ADVANCED_FACE('',(#347),#282,.F.);
#2972=ADVANCED_FACE('',(#348),#2838,.F.);
#2973=ADVANCED_FACE('',(#349),#283,.F.);
#2974=ADVANCED_FACE('',(#350,#180),#2839,.F.);
#2975=ADVANCED_FACE('',(#351),#284,.F.);
#2976=ADVANCED_FACE('',(#352,#181),#2840,.F.);
#2977=ADVANCED_FACE('',(#353),#2841,.T.);
#2978=ADVANCED_FACE('',(#354,#182,#183),#285,.F.);
#2979=ADVANCED_FACE('',(#355),#2842,.T.);
#2980=ADVANCED_FACE('',(#356),#286,.F.);
#2981=ADVANCED_FACE('',(#357),#2843,.T.);
#2982=ADVANCED_FACE('',(#358),#287,.F.);
#2983=ADVANCED_FACE('',(#359),#2844,.T.);
#2984=ADVANCED_FACE('',(#360),#2845,.T.);
#2985=ADVANCED_FACE('',(#361),#2846,.T.);
#2986=ADVANCED_FACE('',(#362,#184),#2847,.T.);
#2987=ADVANCED_FACE('',(#363),#2848,.T.);
#2988=ADVANCED_FACE('',(#364,#185),#2849,.T.);
#2989=ADVANCED_FACE('',(#365,#186,#187,#188,#189),#2850,.T.);
#2990=ADVANCED_FACE('',(#366,#190,#191,#192,#193,#194,#195),#2851,.F.);
#3140=CLOSED_SHELL('',(#2954,#2955,#2956,#2957,#2958,#2959,#2960,#2961,
#2962,#2963,#2964,#2965,#2966,#2967,#2968,#2969,#2970,#2971,#2972,#2973,
#2974,#2975,#2976,#2977,#2978,#2979,#2980,#2981,#2982,#2983,#2984,#2985,
#2986,#2987,#2988,#2989,#2990));
#3310=AXIS2_PLACEMENT_3D('',#4646,#3674,#3675);
#3311=AXIS2_PLACEMENT_3D('',#4647,#3676,#3677);
#3312=AXIS2_PLACEMENT_3D('',#4651,#3679,#3680);
#3313=AXIS2_PLACEMENT_3D('',#4652,#3681,#3682);
#3314=AXIS2_PLACEMENT_3D('',#4655,#3683,#3684);
#3315=AXIS2_PLACEMENT_3D('',#4656,#3685,#3686);
#3316=AXIS2_PLACEMENT_3D('',#4658,#3687,#3688);
#3317=AXIS2_PLACEMENT_3D('',#4661,#3690,#3691);
#3318=AXIS2_PLACEMENT_3D('',#4663,#3692,#3693);
#3319=AXIS2_PLACEMENT_3D('',#4664,#3694,#3695);
#3320=AXIS2_PLACEMENT_3D('',#4665,#3696,#3697);
#3321=AXIS2_PLACEMENT_3D('',#4669,#3699,#3700);
#3322=AXIS2_PLACEMENT_3D('',#4670,#3701,#3702);
#3323=AXIS2_PLACEMENT_3D('',#4674,#3704,#3705);
#3324=AXIS2_PLACEMENT_3D('',#4675,#3706,#3707);
#3325=AXIS2_PLACEMENT_3D('',#4678,#3708,#3709);
#3326=AXIS2_PLACEMENT_3D('',#4681,#3711,#3712);
#3327=AXIS2_PLACEMENT_3D('',#4683,#3713,#3714);
#3328=AXIS2_PLACEMENT_3D('',#4685,#3715,#3716);
#3329=AXIS2_PLACEMENT_3D('',#4687,#3717,#3718);
#3330=AXIS2_PLACEMENT_3D('',#4689,#3719,#3720);
#3331=AXIS2_PLACEMENT_3D('',#4690,#3721,#3722);
#3332=AXIS2_PLACEMENT_3D('',#4691,#3723,#3724);
#3333=AXIS2_PLACEMENT_3D('',#4693,#3725,#3726);
#3334=AXIS2_PLACEMENT_3D('',#4733,#3728,#3729);
#3335=AXIS2_PLACEMENT_3D('',#4735,#3730,#3731);
#3336=AXIS2_PLACEMENT_3D('',#4738,#3733,#3734);
#3337=AXIS2_PLACEMENT_3D('',#4739,#3735,#3736);
#3338=AXIS2_PLACEMENT_3D('',#4740,#3737,#3738);
#3339=AXIS2_PLACEMENT_3D('',#4742,#3739,#3740);
#3340=AXIS2_PLACEMENT_3D('',#4745,#3742,#3743);
#3341=AXIS2_PLACEMENT_3D('',#4746,#3744,#3745);
#3342=AXIS2_PLACEMENT_3D('',#4747,#3746,#3747);
#3343=AXIS2_PLACEMENT_3D('',#4749,#3748,#3749);
#3344=AXIS2_PLACEMENT_3D('',#4752,#3751,#3752);
#3345=AXIS2_PLACEMENT_3D('',#4753,#3753,#3754);
#3346=AXIS2_PLACEMENT_3D('',#4754,#3755,#3756);
#3347=AXIS2_PLACEMENT_3D('',#4756,#3757,#3758);
#3348=AXIS2_PLACEMENT_3D('',#4759,#3760,#3761);
#3349=AXIS2_PLACEMENT_3D('',#4760,#3762,#3763);
#3350=AXIS2_PLACEMENT_3D('',#4761,#3764,#3765);
#3351=AXIS2_PLACEMENT_3D('',#4763,#3766,#3767);
#3352=AXIS2_PLACEMENT_3D('',#4803,#3769,#3770);
#3353=AXIS2_PLACEMENT_3D('',#4805,#3771,#3772);
#3354=AXIS2_PLACEMENT_3D('',#4808,#3774,#3775);
#3355=AXIS2_PLACEMENT_3D('',#4809,#3776,#3777);
#3356=AXIS2_PLACEMENT_3D('',#4810,#3778,#3779);
#3357=AXIS2_PLACEMENT_3D('',#4812,#3780,#3781);
#3358=AXIS2_PLACEMENT_3D('',#4815,#3783,#3784);
#3359=AXIS2_PLACEMENT_3D('',#4816,#3785,#3786);
#3360=AXIS2_PLACEMENT_3D('',#4817,#3787,#3788);
#3361=AXIS2_PLACEMENT_3D('',#4819,#3789,#3790);
#3362=AXIS2_PLACEMENT_3D('',#4822,#3792,#3793);
#3363=AXIS2_PLACEMENT_3D('',#4823,#3794,#3795);
#3364=AXIS2_PLACEMENT_3D('',#4824,#3796,#3797);
#3365=AXIS2_PLACEMENT_3D('',#4826,#3798,#3799);
#3366=AXIS2_PLACEMENT_3D('',#4829,#3801,#3802);
#3367=AXIS2_PLACEMENT_3D('',#4830,#3803,#3804);
#3368=AXIS2_PLACEMENT_3D('',#4831,#3805,#3806);
#3369=AXIS2_PLACEMENT_3D('',#4833,#3808,#3809);
#3370=AXIS2_PLACEMENT_3D('',#4835,#3810,#3811);
#3371=AXIS2_PLACEMENT_3D('',#4841,#3815,#3816);
#3372=AXIS2_PLACEMENT_3D('',#4845,#3818,#3819);
#3373=AXIS2_PLACEMENT_3D('',#4849,#3821,#3822);
#3374=AXIS2_PLACEMENT_3D('',#4853,#3824,#3825);
#3375=AXIS2_PLACEMENT_3D('',#4857,#3828,#3829);
#3376=AXIS2_PLACEMENT_3D('',#4858,#3830,#3831);
#3377=AXIS2_PLACEMENT_3D('',#4859,#3832,#3833);
#3378=AXIS2_PLACEMENT_3D('',#4860,#3834,#3835);
#3379=AXIS2_PLACEMENT_3D('',#4861,#3836,#3837);
#3380=AXIS2_PLACEMENT_3D('',#4863,#3839,#3840);
#3381=AXIS2_PLACEMENT_3D('',#4864,#3841,#3842);
#3382=AXIS2_PLACEMENT_3D('',#4865,#3843,#3844);
#3383=AXIS2_PLACEMENT_3D('',#4868,#3846,#3847);
#3384=AXIS2_PLACEMENT_3D('',#4869,#3848,#3849);
#3385=AXIS2_PLACEMENT_3D('',#4870,#3850,#3851);
#3386=AXIS2_PLACEMENT_3D('',#4871,#3852,#3853);
#3387=AXIS2_PLACEMENT_3D('',#4874,#3855,#3856);
#3388=AXIS2_PLACEMENT_3D('',#4875,#3857,#3858);
#3389=AXIS2_PLACEMENT_3D('',#4876,#3859,#3860);
#3390=AXIS2_PLACEMENT_3D('',#4877,#3861,#3862);
#3391=AXIS2_PLACEMENT_3D('',#4886,#3867,#3868);
#3392=AXIS2_PLACEMENT_3D('',#4892,#3872,#3873);
#3393=AXIS2_PLACEMENT_3D('',#4898,#3877,#3878);
#3394=AXIS2_PLACEMENT_3D('',#4901,#3881,#3882);
#3395=AXIS2_PLACEMENT_3D('',#4902,#3883,#3884);
#3674=DIRECTION('axis',(0.,0.,1.));
#3675=DIRECTION('refdir',(1.,0.,0.));
#3676=DIRECTION('center_axis',(0.,0.,1.));
#3677=DIRECTION('ref_axis',(1.,0.,0.));
#3678=DIRECTION('',(-1.,0.,0.));
#3679=DIRECTION('center_axis',(0.,0.,1.));
#3680=DIRECTION('ref_axis',(1.,0.,0.));
#3681=DIRECTION('center_axis',(0.,0.,1.));
#3682=DIRECTION('ref_axis',(1.,0.,0.));
#3683=DIRECTION('center_axis',(0.707106781186548,0.,-0.707106781186547));
#3684=DIRECTION('ref_axis',(-0.707106781186547,0.,-0.707106781186548));
#3685=DIRECTION('center_axis',(0.707106781186548,0.,-0.707106781186547));
#3686=DIRECTION('ref_axis',(-0.707106781186547,0.,-0.707106781186548));
#3687=DIRECTION('center_axis',(-0.707106781186548,0.,-0.707106781186547));
#3688=DIRECTION('ref_axis',(0.707106781186547,0.,-0.707106781186548));
#3689=DIRECTION('',(0.,0.,1.));
#3690=DIRECTION('center_axis',(0.,0.,-1.));
#3691=DIRECTION('ref_axis',(1.,0.,0.));
#3692=DIRECTION('center_axis',(-0.707106781186548,0.,-0.707106781186547));
#3693=DIRECTION('ref_axis',(0.707106781186547,0.,-0.707106781186548));
#3694=DIRECTION('center_axis',(0.,0.,1.));
#3695=DIRECTION('ref_axis',(1.,0.,0.));
#3696=DIRECTION('center_axis',(0.,0.,1.));
#3697=DIRECTION('ref_axis',(1.,0.,0.));
#3698=DIRECTION('',(1.,0.,0.));
#3699=DIRECTION('center_axis',(0.,0.,1.));
#3700=DIRECTION('ref_axis',(1.,0.,0.));
#3701=DIRECTION('center_axis',(0.,0.,1.));
#3702=DIRECTION('ref_axis',(1.,0.,0.));
#3703=DIRECTION('',(1.,0.,0.));
#3704=DIRECTION('center_axis',(0.,0.,1.));
#3705=DIRECTION('ref_axis',(1.,0.,0.));
#3706=DIRECTION('center_axis',(0.,0.,1.));
#3707=DIRECTION('ref_axis',(1.,0.,0.));
#3708=DIRECTION('center_axis',(-0.707106781186548,0.,-0.707106781186548));
#3709=DIRECTION('ref_axis',(0.707106781186548,0.,-0.707106781186548));
#3710=DIRECTION('',(0.,0.,1.));
#3711=DIRECTION('center_axis',(0.,0.,-1.));
#3712=DIRECTION('ref_axis',(1.,0.,0.));
#3713=DIRECTION('center_axis',(-0.707106781186548,0.,-0.707106781186548));
#3714=DIRECTION('ref_axis',(0.707106781186548,0.,-0.707106781186548));
#3715=DIRECTION('center_axis',(0.,0.,1.));
#3716=DIRECTION('ref_axis',(1.,0.,0.));
#3717=DIRECTION('center_axis',(0.707106781186548,0.,-0.707106781186547));
#3718=DIRECTION('ref_axis',(-0.707106781186547,0.,-0.707106781186548));
#3719=DIRECTION('center_axis',(0.707106781186548,0.,-0.707106781186547));
#3720=DIRECTION('ref_axis',(-0.707106781186547,0.,-0.707106781186548));
#3721=DIRECTION('center_axis',(0.,0.,1.));
#3722=DIRECTION('ref_axis',(1.,0.,0.));
#3723=DIRECTION('center_axis',(0.,0.,1.));
#3724=DIRECTION('ref_axis',(1.,0.,0.));
#3725=DIRECTION('center_axis',(0.,0.,1.));
#3726=DIRECTION('ref_axis',(1.,0.,0.));
#3727=DIRECTION('',(0.,0.,1.));
#3728=DIRECTION('center_axis',(0.,0.,1.));
#3729=DIRECTION('ref_axis',(1.,0.,0.));
#3730=DIRECTION('center_axis',(0.,0.,1.));
#3731=DIRECTION('ref_axis',(1.,0.,0.));
#3732=DIRECTION('',(0.,0.,1.));
#3733=DIRECTION('center_axis',(0.,0.,1.));
#3734=DIRECTION('ref_axis',(1.,0.,0.));
#3735=DIRECTION('center_axis',(0.,0.,1.));
#3736=DIRECTION('ref_axis',(1.,0.,0.));
#3737=DIRECTION('center_axis',(0.,0.,1.));
#3738=DIRECTION('ref_axis',(1.,0.,0.));
#3739=DIRECTION('center_axis',(0.,0.,1.));
#3740=DIRECTION('ref_axis',(1.,0.,0.));
#3741=DIRECTION('',(0.,0.,1.));
#3742=DIRECTION('center_axis',(0.,0.,1.));
#3743=DIRECTION('ref_axis',(1.,0.,0.));
#3744=DIRECTION('center_axis',(0.,0.,1.));
#3745=DIRECTION('ref_axis',(1.,0.,0.));
#3746=DIRECTION('center_axis',(0.,0.,1.));
#3747=DIRECTION('ref_axis',(1.,0.,0.));
#3748=DIRECTION('center_axis',(0.,0.,1.));
#3749=DIRECTION('ref_axis',(1.,0.,0.));
#3750=DIRECTION('',(0.,0.,1.));
#3751=DIRECTION('center_axis',(0.,0.,1.));
#3752=DIRECTION('ref_axis',(1.,0.,0.));
#3753=DIRECTION('center_axis',(0.,0.,1.));
#3754=DIRECTION('ref_axis',(1.,0.,0.));
#3755=DIRECTION('center_axis',(0.,0.,1.));
#3756=DIRECTION('ref_axis',(1.,0.,0.));
#3757=DIRECTION('center_axis',(0.,0.,1.));
#3758=DIRECTION('ref_axis',(1.,0.,0.));
#3759=DIRECTION('',(0.,0.,1.));
#3760=DIRECTION('center_axis',(0.,0.,1.));
#3761=DIRECTION('ref_axis',(1.,0.,0.));
#3762=DIRECTION('center_axis',(0.,0.,1.));
#3763=DIRECTION('ref_axis',(1.,0.,0.));
#3764=DIRECTION('center_axis',(0.,0.,1.));
#3765=DIRECTION('ref_axis',(1.,0.,0.));
#3766=DIRECTION('center_axis',(0.,0.,1.));
#3767=DIRECTION('ref_axis',(1.,0.,0.));
#3768=DIRECTION('',(0.,0.,1.));
#3769=DIRECTION('center_axis',(0.,0.,1.));
#3770=DIRECTION('ref_axis',(1.,0.,0.));
#3771=DIRECTION('center_axis',(0.,0.,1.));
#3772=DIRECTION('ref_axis',(1.,0.,0.));
#3773=DIRECTION('',(0.,0.,1.));
#3774=DIRECTION('center_axis',(0.,0.,1.));
#3775=DIRECTION('ref_axis',(1.,0.,0.));
#3776=DIRECTION('center_axis',(0.,0.,1.));
#3777=DIRECTION('ref_axis',(1.,0.,0.));
#3778=DIRECTION('center_axis',(0.,0.,1.));
#3779=DIRECTION('ref_axis',(1.,0.,0.));
#3780=DIRECTION('center_axis',(0.,0.,1.));
#3781=DIRECTION('ref_axis',(1.,0.,0.));
#3782=DIRECTION('',(0.,0.,1.));
#3783=DIRECTION('center_axis',(0.,0.,1.));
#3784=DIRECTION('ref_axis',(1.,0.,0.));
#3785=DIRECTION('center_axis',(0.,0.,1.));
#3786=DIRECTION('ref_axis',(1.,0.,0.));
#3787=DIRECTION('center_axis',(0.,0.,1.));
#3788=DIRECTION('ref_axis',(1.,0.,0.));
#3789=DIRECTION('center_axis',(0.,0.,1.));
#3790=DIRECTION('ref_axis',(1.,0.,0.));
#3791=DIRECTION('',(0.,0.,1.));
#3792=DIRECTION('center_axis',(0.,0.,1.));
#3793=DIRECTION('ref_axis',(1.,0.,0.));
#3794=DIRECTION('center_axis',(0.,0.,1.));
#3795=DIRECTION('ref_axis',(1.,0.,0.));
#3796=DIRECTION('center_axis',(0.,0.,1.));
#3797=DIRECTION('ref_axis',(1.,0.,0.));
#3798=DIRECTION('center_axis',(0.,0.,1.));
#3799=DIRECTION('ref_axis',(1.,0.,0.));
#3800=DIRECTION('',(0.,0.,1.));
#3801=DIRECTION('center_axis',(0.,0.,1.));
#3802=DIRECTION('ref_axis',(1.,0.,0.));
#3803=DIRECTION('center_axis',(0.,0.,1.));
#3804=DIRECTION('ref_axis',(1.,0.,0.));
#3805=DIRECTION('center_axis',(0.,0.,1.));
#3806=DIRECTION('ref_axis',(1.,0.,0.));
#3807=DIRECTION('',(1.,0.,0.));
#3808=DIRECTION('center_axis',(1.,0.,0.));
#3809=DIRECTION('ref_axis',(0.,0.,-1.));
#3810=DIRECTION('center_axis',(1.,0.,0.));
#3811=DIRECTION('ref_axis',(0.,0.,-1.));
#3812=DIRECTION('',(1.,0.,0.));
#3813=DIRECTION('',(-1.,0.,0.));
#3814=DIRECTION('',(1.,0.,0.));
#3815=DIRECTION('center_axis',(-0.707106781186548,0.,-0.707106781186547));
#3816=DIRECTION('ref_axis',(0.707106781186547,0.,-0.707106781186548));
#3817=DIRECTION('',(-1.,0.,0.));
#3818=DIRECTION('center_axis',(0.707106781186548,0.,-0.707106781186547));
#3819=DIRECTION('ref_axis',(-0.707106781186547,0.,-0.707106781186548));
#3820=DIRECTION('',(1.,0.,0.));
#3821=DIRECTION('center_axis',(-0.707106781186548,0.,-0.707106781186547));
#3822=DIRECTION('ref_axis',(0.707106781186547,0.,-0.707106781186548));
#3823=DIRECTION('',(-1.,0.,0.));
#3824=DIRECTION('center_axis',(0.707106781186548,0.,-0.707106781186547));
#3825=DIRECTION('ref_axis',(-0.707106781186547,0.,-0.707106781186548));
#3826=DIRECTION('',(1.,0.,0.));
#3827=DIRECTION('',(1.,0.,0.));
#3828=DIRECTION('center_axis',(-1.,0.,0.));
#3829=DIRECTION('ref_axis',(0.,0.,-1.));
#3830=DIRECTION('center_axis',(0.707106781186548,0.,-0.707106781186547));
#3831=DIRECTION('ref_axis',(-0.707106781186547,0.,-0.707106781186548));
#3832=DIRECTION('center_axis',(-0.707106781186548,0.,-0.707106781186547));
#3833=DIRECTION('ref_axis',(0.707106781186547,0.,-0.707106781186548));
#3834=DIRECTION('center_axis',(0.707106781186548,0.,-0.707106781186547));
#3835=DIRECTION('ref_axis',(-0.707106781186547,0.,-0.707106781186548));
#3836=DIRECTION('center_axis',(-0.707106781186548,0.,-0.707106781186547));
#3837=DIRECTION('ref_axis',(0.707106781186547,0.,-0.707106781186548));
#3838=DIRECTION('',(1.,0.,0.));
#3839=DIRECTION('center_axis',(0.,0.,1.));
#3840=DIRECTION('ref_axis',(1.,0.,0.));
#3841=DIRECTION('center_axis',(0.,0.,1.));
#3842=DIRECTION('ref_axis',(1.,0.,0.));
#3843=DIRECTION('center_axis',(0.,0.,1.));
#3844=DIRECTION('ref_axis',(1.,0.,0.));
#3845=DIRECTION('',(0.,0.,1.));
#3846=DIRECTION('center_axis',(0.,0.,-1.));
#3847=DIRECTION('ref_axis',(1.,0.,0.));
#3848=DIRECTION('center_axis',(0.,0.,1.));
#3849=DIRECTION('ref_axis',(1.,0.,0.));
#3850=DIRECTION('center_axis',(0.,0.,1.));
#3851=DIRECTION('ref_axis',(1.,0.,0.));
#3852=DIRECTION('center_axis',(0.,0.,1.));
#3853=DIRECTION('ref_axis',(1.,0.,0.));
#3854=DIRECTION('',(0.,0.,1.));
#3855=DIRECTION('center_axis',(0.,0.,-1.));
#3856=DIRECTION('ref_axis',(1.,0.,0.));
#3857=DIRECTION('center_axis',(0.,0.,1.));
#3858=DIRECTION('ref_axis',(1.,0.,0.));
#3859=DIRECTION('center_axis',(0.,0.,1.));
#3860=DIRECTION('ref_axis',(1.,0.,0.));
#3861=DIRECTION('center_axis',(0.,1.,0.));
#3862=DIRECTION('ref_axis',(-1.,0.,0.));
#3863=DIRECTION('',(-1.,0.,0.));
#3864=DIRECTION('',(0.,0.,1.));
#3865=DIRECTION('',(-1.,0.,0.));
#3866=DIRECTION('',(0.,0.,1.));
#3867=DIRECTION('center_axis',(1.,0.,0.));
#3868=DIRECTION('ref_axis',(0.,1.,0.));
#3869=DIRECTION('',(0.,1.,0.));
#3870=DIRECTION('',(0.,1.,0.));
#3871=DIRECTION('',(0.,0.,1.));
#3872=DIRECTION('center_axis',(0.,-1.,0.));
#3873=DIRECTION('ref_axis',(1.,0.,0.));
#3874=DIRECTION('',(1.,0.,0.));
#3875=DIRECTION('',(1.,0.,0.));
#3876=DIRECTION('',(0.,0.,1.));
#3877=DIRECTION('center_axis',(-1.,0.,0.));
#3878=DIRECTION('ref_axis',(0.,-1.,0.));
#3879=DIRECTION('',(0.,-1.,0.));
#3880=DIRECTION('',(0.,-1.,0.));
#3881=DIRECTION('center_axis',(0.,0.,1.));
#3882=DIRECTION('ref_axis',(1.,0.,0.));
#3883=DIRECTION('center_axis',(0.,0.,1.));
#3884=DIRECTION('ref_axis',(1.,0.,0.));
#4646=CARTESIAN_POINT('',(0.,0.,0.));
#4647=CARTESIAN_POINT('Origin',(3.75,0.,3.8));
#4648=CARTESIAN_POINT('',(4.05,-0.615812471455394,3.8));
#4649=CARTESIAN_POINT('',(3.45,-0.615812471455394,3.8));
#4650=CARTESIAN_POINT('',(-5.5,-0.615812471455394,3.8));
#4651=CARTESIAN_POINT('Origin',(3.75,0.,3.8));
#4652=CARTESIAN_POINT('Origin',(3.75,0.,3.8));
#4653=CARTESIAN_POINT('',(4.05,0.615812471455394,3.8));
#4654=CARTESIAN_POINT('',(4.435,-8.38883057415936E-17,4.185));
#4655=CARTESIAN_POINT('Origin',(3.75,0.,3.5));
#4656=CARTESIAN_POINT('Origin',(3.75,0.,3.5));
#4657=CARTESIAN_POINT('',(3.065,-8.38883057415936E-17,4.185));
#4658=CARTESIAN_POINT('Origin',(3.75,0.,3.5));
#4659=CARTESIAN_POINT('',(3.065,8.38883057415936E-17,5.));
#4660=CARTESIAN_POINT('',(3.065,-8.38883057415936E-17,3.8));
#4661=CARTESIAN_POINT('Origin',(3.75,0.,5.));
#4662=CARTESIAN_POINT('',(3.45,0.615812471455394,3.8));
#4663=CARTESIAN_POINT('Origin',(3.75,0.,3.5));
#4664=CARTESIAN_POINT('Origin',(3.75,0.,3.8));
#4665=CARTESIAN_POINT('Origin',(1.25,0.,3.8));
#4666=CARTESIAN_POINT('',(0.95,0.615812471455394,3.8));
#4667=CARTESIAN_POINT('',(1.55,0.615812471455394,3.8));
#4668=CARTESIAN_POINT('',(-5.5,0.615812471455394,3.8));
#4669=CARTESIAN_POINT('Origin',(1.25,0.,3.8));
#4670=CARTESIAN_POINT('Origin',(-1.25,0.,3.8));
#4671=CARTESIAN_POINT('',(-1.55,0.615812471455394,3.8));
#4672=CARTESIAN_POINT('',(-0.95,0.615812471455394,3.8));
#4673=CARTESIAN_POINT('',(-5.5,0.615812471455394,3.8));
#4674=CARTESIAN_POINT('Origin',(-1.25,0.,3.8));
#4675=CARTESIAN_POINT('Origin',(-3.75,0.,3.8));
#4676=CARTESIAN_POINT('',(-4.05,-0.615812471455394,3.8));
#4677=CARTESIAN_POINT('',(-4.435,-8.38883057415937E-17,4.185));
#4678=CARTESIAN_POINT('Origin',(-3.75,0.,3.5));
#4679=CARTESIAN_POINT('',(-4.435,8.38883057415937E-17,5.));
#4680=CARTESIAN_POINT('',(-4.435,-8.38883057415937E-17,3.8));
#4681=CARTESIAN_POINT('Origin',(-3.75,0.,5.));
#4682=CARTESIAN_POINT('',(-4.05,0.615812471455394,3.8));
#4683=CARTESIAN_POINT('Origin',(-3.75,0.,3.5));
#4684=CARTESIAN_POINT('',(-3.45,0.615812471455394,3.8));
#4685=CARTESIAN_POINT('Origin',(-3.75,0.,3.8));
#4686=CARTESIAN_POINT('',(-3.065,-8.38883057415936E-17,4.185));
#4687=CARTESIAN_POINT('Origin',(-3.75,0.,3.5));
#4688=CARTESIAN_POINT('',(-3.45,-0.615812471455394,3.8));
#4689=CARTESIAN_POINT('Origin',(-3.75,0.,3.5));
#4690=CARTESIAN_POINT('Origin',(-3.75,0.,3.8));
#4691=CARTESIAN_POINT('Origin',(4.5,0.,0.9));
#4692=CARTESIAN_POINT('',(4.295,-2.51052593825207E-17,2.));
#4693=CARTESIAN_POINT('Origin',(4.5,0.,2.));
#4694=CARTESIAN_POINT('',(4.295,-5.61373578735315E-18,2.815));
#4695=CARTESIAN_POINT('',(4.295,-2.51052593825207E-17,0.9));
#4696=CARTESIAN_POINT('',(4.5,-0.205,2.84639461446527));
#4697=CARTESIAN_POINT('Ctrl Pts',(4.5,-0.205,2.84639461446527));
#4698=CARTESIAN_POINT('Ctrl Pts',(4.4740836410313,-0.205,2.84639461446527));
#4699=CARTESIAN_POINT('Ctrl Pts',(4.4465572469413,-0.199787945222222,2.84469184063064));
#4700=CARTESIAN_POINT('Ctrl Pts',(4.3961018032059,-0.178819800999948,2.83866235487196));
#4701=CARTESIAN_POINT('Ctrl Pts',(4.37315766716202,-0.163071447448502,2.83443540996919));
#4702=CARTESIAN_POINT('Ctrl Pts',(4.33693389431385,-0.12684767460033,2.82659225921127));
#4703=CARTESIAN_POINT('Ctrl Pts',(4.32118140385364,-0.103901367097065,2.82244952053683));
#4704=CARTESIAN_POINT('Ctrl Pts',(4.3002102058406,-0.0534380328956992,2.81661539166144));
#4705=CARTESIAN_POINT('Ctrl Pts',(4.295,-0.0259087165500479,2.815));
#4706=CARTESIAN_POINT('Ctrl Pts',(4.295,-6.24500451351651E-17,2.815));
#4707=CARTESIAN_POINT('Ctrl Pts',(4.295,2.08166817117217E-17,2.815));
#4708=CARTESIAN_POINT('Ctrl Pts',(4.295,0.0259087165500478,2.815));
#4709=CARTESIAN_POINT('Ctrl Pts',(4.3002102058406,0.0534380328956991,2.81661539166144));
#4710=CARTESIAN_POINT('Ctrl Pts',(4.32118140385364,0.103901367097065,2.82244952053683));
#4711=CARTESIAN_POINT('Ctrl Pts',(4.33693389431385,0.12684767460033,2.82659225921127));
#4712=CARTESIAN_POINT('Ctrl Pts',(4.37315766716202,0.163071447448502,2.83443540996919));
#4713=CARTESIAN_POINT('Ctrl Pts',(4.3961018032059,0.178819800999948,2.83866235487196));
#4714=CARTESIAN_POINT('Ctrl Pts',(4.4465572469413,0.199787945222222,2.84469184063064));
#4715=CARTESIAN_POINT('Ctrl Pts',(4.47408364103131,0.205,2.84639461446527));
#4716=CARTESIAN_POINT('Ctrl Pts',(4.52591635896869,0.205,2.84639461446527));
#4717=CARTESIAN_POINT('Ctrl Pts',(4.5534427530587,0.199787945222222,2.84469184063064));
#4718=CARTESIAN_POINT('Ctrl Pts',(4.6038981967941,0.178819800999948,2.83866235487196));
#4719=CARTESIAN_POINT('Ctrl Pts',(4.62684233283798,0.163071447448502,2.83443540996919));
#4720=CARTESIAN_POINT('Ctrl Pts',(4.66306610568615,0.12684767460033,2.82659225921127));
#4721=CARTESIAN_POINT('Ctrl Pts',(4.67881859614636,0.103901367097065,2.82244952053683));
#4722=CARTESIAN_POINT('Ctrl Pts',(4.6997897941594,0.0534380328956992,2.81661539166144));
#4723=CARTESIAN_POINT('Ctrl Pts',(4.705,0.0259087165500479,2.815));
#4724=CARTESIAN_POINT('Ctrl Pts',(4.705,-0.0259087165500477,2.815));
#4725=CARTESIAN_POINT('Ctrl Pts',(4.6997897941594,-0.0534380328956993,2.81661539166144));
#4726=CARTESIAN_POINT('Ctrl Pts',(4.67881859614636,-0.103901367097066,2.82244952053683));
#4727=CARTESIAN_POINT('Ctrl Pts',(4.66306610568615,-0.12684767460033,2.82659225921127));
#4728=CARTESIAN_POINT('Ctrl Pts',(4.62684233283798,-0.163071447448502,2.83443540996919));
#4729=CARTESIAN_POINT('Ctrl Pts',(4.6038981967941,-0.178819800999948,2.83866235487196));
#4730=CARTESIAN_POINT('Ctrl Pts',(4.5534427530587,-0.199787945222222,2.84469184063064));
#4731=CARTESIAN_POINT('Ctrl Pts',(4.5259163589687,-0.205,2.84639461446527));
#4732=CARTESIAN_POINT('Ctrl Pts',(4.5,-0.205,2.84639461446527));
#4733=CARTESIAN_POINT('Origin',(4.5,-1.2,1.9));
#4734=CARTESIAN_POINT('',(4.25,-1.2,2.1));
#4735=CARTESIAN_POINT('Origin',(4.5,-1.2,2.1));
#4736=CARTESIAN_POINT('',(4.25,-1.2,4.7));
#4737=CARTESIAN_POINT('',(4.25,-1.2,1.9));
#4738=CARTESIAN_POINT('Origin',(4.5,-1.2,4.7));
#4739=CARTESIAN_POINT('Origin',(4.5,-1.2,4.7));
#4740=CARTESIAN_POINT('Origin',(4.5,1.2,1.9));
#4741=CARTESIAN_POINT('',(4.25,1.2,2.1));
#4742=CARTESIAN_POINT('Origin',(4.5,1.2,2.1));
#4743=CARTESIAN_POINT('',(4.25,1.2,4.7));
#4744=CARTESIAN_POINT('',(4.25,1.2,1.9));
#4745=CARTESIAN_POINT('Origin',(4.5,1.2,4.7));
#4746=CARTESIAN_POINT('Origin',(4.5,1.2,4.7));
#4747=CARTESIAN_POINT('Origin',(4.5,-1.2,0.9));
#4748=CARTESIAN_POINT('',(4.17,-1.2,2.));
#4749=CARTESIAN_POINT('Origin',(4.5,-1.2,2.));
#4750=CARTESIAN_POINT('',(4.17,-1.2,2.1));
#4751=CARTESIAN_POINT('',(4.17,-1.2,0.9));
#4752=CARTESIAN_POINT('Origin',(4.5,-1.2,2.1));
#4753=CARTESIAN_POINT('Origin',(4.5,-1.2,2.1));
#4754=CARTESIAN_POINT('Origin',(4.5,1.2,0.9));
#4755=CARTESIAN_POINT('',(4.17,1.2,2.));
#4756=CARTESIAN_POINT('Origin',(4.5,1.2,2.));
#4757=CARTESIAN_POINT('',(4.17,1.2,2.1));
#4758=CARTESIAN_POINT('',(4.17,1.2,0.9));
#4759=CARTESIAN_POINT('Origin',(4.5,1.2,2.1));
#4760=CARTESIAN_POINT('Origin',(4.5,1.2,2.1));
#4761=CARTESIAN_POINT('Origin',(-4.5,0.,0.9));
#4762=CARTESIAN_POINT('',(-4.705,-2.51052593825207E-17,2.));
#4763=CARTESIAN_POINT('Origin',(-4.5,0.,2.));
#4764=CARTESIAN_POINT('',(-4.705,-2.98998644510284E-17,2.815));
#4765=CARTESIAN_POINT('',(-4.705,-2.51052593825207E-17,0.9));
#4766=CARTESIAN_POINT('',(-4.5,-0.205,2.84639461446527));
#4767=CARTESIAN_POINT('Ctrl Pts',(-4.5,-0.205,2.84639461446527));
#4768=CARTESIAN_POINT('Ctrl Pts',(-4.52591635896869,-0.205,2.84639461446527));
#4769=CARTESIAN_POINT('Ctrl Pts',(-4.5534427530587,-0.199787945222222,2.84469184063064));
#4770=CARTESIAN_POINT('Ctrl Pts',(-4.6038981967941,-0.178819800999948,2.83866235487196));
#4771=CARTESIAN_POINT('Ctrl Pts',(-4.62684233283798,-0.163071447448502,
2.83443540996919));
#4772=CARTESIAN_POINT('Ctrl Pts',(-4.66306610568615,-0.12684767460033,2.82659225921127));
#4773=CARTESIAN_POINT('Ctrl Pts',(-4.67881859614636,-0.103901367097065,
2.82244952053683));
#4774=CARTESIAN_POINT('Ctrl Pts',(-4.6997897941594,-0.0534380328956992,
2.81661539166144));
#4775=CARTESIAN_POINT('Ctrl Pts',(-4.705,-0.0259087165500478,2.815));
#4776=CARTESIAN_POINT('Ctrl Pts',(-4.705,-1.38777878078145E-17,2.815));
#4777=CARTESIAN_POINT('Ctrl Pts',(-4.705,-2.77555756156289E-17,2.815));
#4778=CARTESIAN_POINT('Ctrl Pts',(-4.705,0.0259087165500478,2.815));
#4779=CARTESIAN_POINT('Ctrl Pts',(-4.6997897941594,0.0534380328956991,2.81661539166144));
#4780=CARTESIAN_POINT('Ctrl Pts',(-4.67881859614636,0.103901367097065,2.82244952053683));
#4781=CARTESIAN_POINT('Ctrl Pts',(-4.66306610568615,0.12684767460033,2.82659225921127));
#4782=CARTESIAN_POINT('Ctrl Pts',(-4.62684233283798,0.163071447448502,2.83443540996919));
#4783=CARTESIAN_POINT('Ctrl Pts',(-4.6038981967941,0.178819800999948,2.83866235487196));
#4784=CARTESIAN_POINT('Ctrl Pts',(-4.5534427530587,0.199787945222222,2.84469184063064));
#4785=CARTESIAN_POINT('Ctrl Pts',(-4.52591635896869,0.205,2.84639461446527));
#4786=CARTESIAN_POINT('Ctrl Pts',(-4.47408364103131,0.205,2.84639461446527));
#4787=CARTESIAN_POINT('Ctrl Pts',(-4.4465572469413,0.199787945222222,2.84469184063064));
#4788=CARTESIAN_POINT('Ctrl Pts',(-4.3961018032059,0.178819800999948,2.83866235487196));
#4789=CARTESIAN_POINT('Ctrl Pts',(-4.37315766716202,0.163071447448502,2.83443540996919));
#4790=CARTESIAN_POINT('Ctrl Pts',(-4.33693389431385,0.12684767460033,2.82659225921127));
#4791=CARTESIAN_POINT('Ctrl Pts',(-4.32118140385364,0.103901367097065,2.82244952053683));
#4792=CARTESIAN_POINT('Ctrl Pts',(-4.3002102058406,0.0534380328956992,2.81661539166144));
#4793=CARTESIAN_POINT('Ctrl Pts',(-4.295,0.0259087165500479,2.815));
#4794=CARTESIAN_POINT('Ctrl Pts',(-4.295,-0.0259087165500477,2.815));
#4795=CARTESIAN_POINT('Ctrl Pts',(-4.3002102058406,-0.0534380328956982,
2.81661539166144));
#4796=CARTESIAN_POINT('Ctrl Pts',(-4.32118140385364,-0.103901367097065,
2.82244952053683));
#4797=CARTESIAN_POINT('Ctrl Pts',(-4.33693389431385,-0.12684767460033,2.82659225921127));
#4798=CARTESIAN_POINT('Ctrl Pts',(-4.37315766716202,-0.163071447448502,
2.83443540996919));
#4799=CARTESIAN_POINT('Ctrl Pts',(-4.3961018032059,-0.178819800999948,2.83866235487196));
#4800=CARTESIAN_POINT('Ctrl Pts',(-4.4465572469413,-0.199787945222222,2.84469184063064));
#4801=CARTESIAN_POINT('Ctrl Pts',(-4.47408364103131,-0.205,2.84639461446527));
#4802=CARTESIAN_POINT('Ctrl Pts',(-4.5,-0.205,2.84639461446527));
#4803=CARTESIAN_POINT('Origin',(-4.5,-1.2,1.9));
#4804=CARTESIAN_POINT('',(-4.75,-1.2,2.1));
#4805=CARTESIAN_POINT('Origin',(-4.5,-1.2,2.1));
#4806=CARTESIAN_POINT('',(-4.75,-1.2,4.7));
#4807=CARTESIAN_POINT('',(-4.75,-1.2,1.9));
#4808=CARTESIAN_POINT('Origin',(-4.5,-1.2,4.7));
#4809=CARTESIAN_POINT('Origin',(-4.5,-1.2,4.7));
#4810=CARTESIAN_POINT('Origin',(-4.5,1.2,1.9));
#4811=CARTESIAN_POINT('',(-4.75,1.2,2.1));
#4812=CARTESIAN_POINT('Origin',(-4.5,1.2,2.1));
#4813=CARTESIAN_POINT('',(-4.75,1.2,4.7));
#4814=CARTESIAN_POINT('',(-4.75,1.2,1.9));
#4815=CARTESIAN_POINT('Origin',(-4.5,1.2,4.7));
#4816=CARTESIAN_POINT('Origin',(-4.5,1.2,4.7));
#4817=CARTESIAN_POINT('Origin',(-4.5,-1.2,0.9));
#4818=CARTESIAN_POINT('',(-4.83,-1.2,2.));
#4819=CARTESIAN_POINT('Origin',(-4.5,-1.2,2.));
#4820=CARTESIAN_POINT('',(-4.83,-1.2,2.1));
#4821=CARTESIAN_POINT('',(-4.83,-1.2,0.9));
#4822=CARTESIAN_POINT('Origin',(-4.5,-1.2,2.1));
#4823=CARTESIAN_POINT('Origin',(-4.5,-1.2,2.1));
#4824=CARTESIAN_POINT('Origin',(-4.5,1.2,0.9));
#4825=CARTESIAN_POINT('',(-4.83,1.2,2.));
#4826=CARTESIAN_POINT('Origin',(-4.5,1.2,2.));
#4827=CARTESIAN_POINT('',(-4.83,1.2,2.1));
#4828=CARTESIAN_POINT('',(-4.83,1.2,0.9));
#4829=CARTESIAN_POINT('Origin',(-4.5,1.2,2.1));
#4830=CARTESIAN_POINT('Origin',(-4.5,1.2,2.1));
#4831=CARTESIAN_POINT('Origin',(3.75,0.,3.8));
#4832=CARTESIAN_POINT('',(-5.5,0.615812471455394,3.8));
#4833=CARTESIAN_POINT('Origin',(4.1,0.,3.5));
#4834=CARTESIAN_POINT('',(-5.5,-8.38883057415937E-17,4.185));
#4835=CARTESIAN_POINT('Origin',(-5.5,0.,3.5));
#4836=CARTESIAN_POINT('',(4.1,-8.38883057415937E-17,4.185));
#4837=CARTESIAN_POINT('',(-5.5,-0.615812471455394,3.8));
#4838=CARTESIAN_POINT('',(-1.935,-8.38883057415937E-17,4.185));
#4839=CARTESIAN_POINT('',(4.1,-8.38883057415937E-17,4.185));
#4840=CARTESIAN_POINT('',(-1.55,-0.615812471455394,3.8));
#4841=CARTESIAN_POINT('Origin',(-1.25,0.,3.5));
#4842=CARTESIAN_POINT('',(-0.95,-0.615812471455394,3.8));
#4843=CARTESIAN_POINT('',(-5.5,-0.615812471455394,3.8));
#4844=CARTESIAN_POINT('',(-0.565000000000001,-8.38883057415936E-17,4.185));
#4845=CARTESIAN_POINT('Origin',(-1.25,0.,3.5));
#4846=CARTESIAN_POINT('',(0.565000000000001,-8.38883057415936E-17,4.185));
#4847=CARTESIAN_POINT('',(4.1,-8.38883057415937E-17,4.185));
#4848=CARTESIAN_POINT('',(0.95,-0.615812471455394,3.8));
#4849=CARTESIAN_POINT('Origin',(1.25,0.,3.5));
#4850=CARTESIAN_POINT('',(1.55,-0.615812471455394,3.8));
#4851=CARTESIAN_POINT('',(-5.5,-0.615812471455394,3.8));
#4852=CARTESIAN_POINT('',(1.935,-8.38883057415936E-17,4.185));
#4853=CARTESIAN_POINT('Origin',(1.25,0.,3.5));
#4854=CARTESIAN_POINT('',(4.1,-8.38883057415937E-17,4.185));
#4855=CARTESIAN_POINT('',(5.5,8.38883057415937E-17,4.185));
#4856=CARTESIAN_POINT('',(4.1,-8.38883057415937E-17,4.185));
#4857=CARTESIAN_POINT('Origin',(5.5,0.,3.5));
#4858=CARTESIAN_POINT('Origin',(1.25,0.,3.5));
#4859=CARTESIAN_POINT('Origin',(1.25,0.,3.5));
#4860=CARTESIAN_POINT('Origin',(-1.25,0.,3.5));
#4861=CARTESIAN_POINT('Origin',(-1.25,0.,3.5));
#4862=CARTESIAN_POINT('',(-5.5,0.615812471455394,3.8));
#4863=CARTESIAN_POINT('Origin',(1.25,0.,3.8));
#4864=CARTESIAN_POINT('Origin',(1.25,0.,3.8));
#4865=CARTESIAN_POINT('Origin',(1.25,0.,3.8));
#4866=CARTESIAN_POINT('',(0.565,8.38883057415937E-17,5.));
#4867=CARTESIAN_POINT('',(0.565,-8.38883057415937E-17,3.8));
#4868=CARTESIAN_POINT('Origin',(1.25,0.,5.));
#4869=CARTESIAN_POINT('Origin',(-1.25,0.,3.8));
#4870=CARTESIAN_POINT('Origin',(-1.25,0.,3.8));
#4871=CARTESIAN_POINT('Origin',(-1.25,0.,3.8));
#4872=CARTESIAN_POINT('',(-1.935,8.38883057415937E-17,5.));
#4873=CARTESIAN_POINT('',(-1.935,-8.38883057415937E-17,3.8));
#4874=CARTESIAN_POINT('Origin',(-1.25,0.,5.));
#4875=CARTESIAN_POINT('Origin',(-3.75,0.,3.8));
#4876=CARTESIAN_POINT('Origin',(-3.75,0.,3.8));
#4877=CARTESIAN_POINT('Origin',(5.5,2.,2.));
#4878=CARTESIAN_POINT('',(5.5,2.,2.));
#4879=CARTESIAN_POINT('',(-5.5,2.,2.));
#4880=CARTESIAN_POINT('',(5.5,2.,2.));
#4881=CARTESIAN_POINT('',(-5.5,2.,5.));
#4882=CARTESIAN_POINT('',(-5.5,2.,2.));
#4883=CARTESIAN_POINT('',(5.5,2.,5.));
#4884=CARTESIAN_POINT('',(5.5,2.,5.));
#4885=CARTESIAN_POINT('',(5.5,2.,2.));
#4886=CARTESIAN_POINT('Origin',(5.5,-2.,2.));
#4887=CARTESIAN_POINT('',(5.5,-2.,2.));
#4888=CARTESIAN_POINT('',(5.5,-2.,2.));
#4889=CARTESIAN_POINT('',(5.5,-2.,5.));
#4890=CARTESIAN_POINT('',(5.5,-2.,5.));
#4891=CARTESIAN_POINT('',(5.5,-2.,2.));
#4892=CARTESIAN_POINT('Origin',(-5.5,-2.,2.));
#4893=CARTESIAN_POINT('',(-5.5,-2.,2.));
#4894=CARTESIAN_POINT('',(-5.5,-2.,2.));
#4895=CARTESIAN_POINT('',(-5.5,-2.,5.));
#4896=CARTESIAN_POINT('',(-5.5,-2.,5.));
#4897=CARTESIAN_POINT('',(-5.5,-2.,2.));
#4898=CARTESIAN_POINT('Origin',(-5.5,2.,2.));
#4899=CARTESIAN_POINT('',(-5.5,2.,2.));
#4900=CARTESIAN_POINT('',(-5.5,2.,5.));
#4901=CARTESIAN_POINT('Origin',(0.,0.,5.));
#4902=CARTESIAN_POINT('Origin',(0.,0.,2.));
#5606=UNCERTAINTY_MEASURE_WITH_UNIT(LENGTH_MEASURE(0.001),#5639,
'DISTANCE_ACCURACY_VALUE',
'Maximum model space distance between geometric entities at asserted c
onnectivities');
#5621=UNCERTAINTY_MEASURE_WITH_UNIT(LENGTH_MEASURE(0.001),#5639,
'DISTANCE_ACCURACY_VALUE',
'Maximum model space distance between geometric entities at asserted c
onnectivities');
#5623=(
GEOMETRIC_REPRESENTATION_CONTEXT(3)
GLOBAL_UNCERTAINTY_ASSIGNED_CONTEXT((#5606))
GLOBAL_UNIT_ASSIGNED_CONTEXT((#5639,#5641,#5642))
REPRESENTATION_CONTEXT('','3D')
);
#5638=(
GEOMETRIC_REPRESENTATION_CONTEXT(3)
GLOBAL_UNCERTAINTY_ASSIGNED_CONTEXT((#5621))
GLOBAL_UNIT_ASSIGNED_CONTEXT((#5639,#5641,#5642))
REPRESENTATION_CONTEXT('','3D')
);
#5639=(
LENGTH_UNIT()
NAMED_UNIT(*)
SI_UNIT(.CENTI.,.METRE.)
);
#5641=(
NAMED_UNIT(*)
PLANE_ANGLE_UNIT()
SI_UNIT($,.RADIAN.)
);
#5642=(
NAMED_UNIT(*)
SI_UNIT($,.STERADIAN.)
SOLID_ANGLE_UNIT()
);
#5644=SHAPE_DEFINITION_REPRESENTATION(#5660,#5701);
#5660=PRODUCT_DEFINITION_SHAPE('',$,#5718);
#5701=SHAPE_REPRESENTATION('',(#3310),#5623);
#5716=PRODUCT_DEFINITION_CONTEXT('part definition',#5766,'design');
#5718=PRODUCT_DEFINITION('Manifold block','Manifold block',#5734,
#5716);
#5734=PRODUCT_DEFINITION_FORMATION('',$,#5769);
#5766=APPLICATION_CONTEXT(
'Core Data for Automotive Mechanical Design Process');
#5767=PRODUCT_CONTEXT('part definition',#5766,'mechanical');
#5769=PRODUCT('Manifold block','Manifold block',
'Manifold block',(#5767));
#5833=COLOUR_RGB('Dark Blue',0.08,0.2,0.34);
#5834=FILL_AREA_STYLE_COLOUR('',#5833);
#5835=FILL_AREA_STYLE('',(#5834));
#5836=SURFACE_STYLE_FILL_AREA(#5835);
#5837=SURFACE_SIDE_STYLE('',(#5836));
#5838=SURFACE_STYLE_USAGE(.BOTH.,#5837);
#5839=PRESENTATION_STYLE_ASSIGNMENT((#5838));
ENDSEC;
END-ISO-10303-21;
